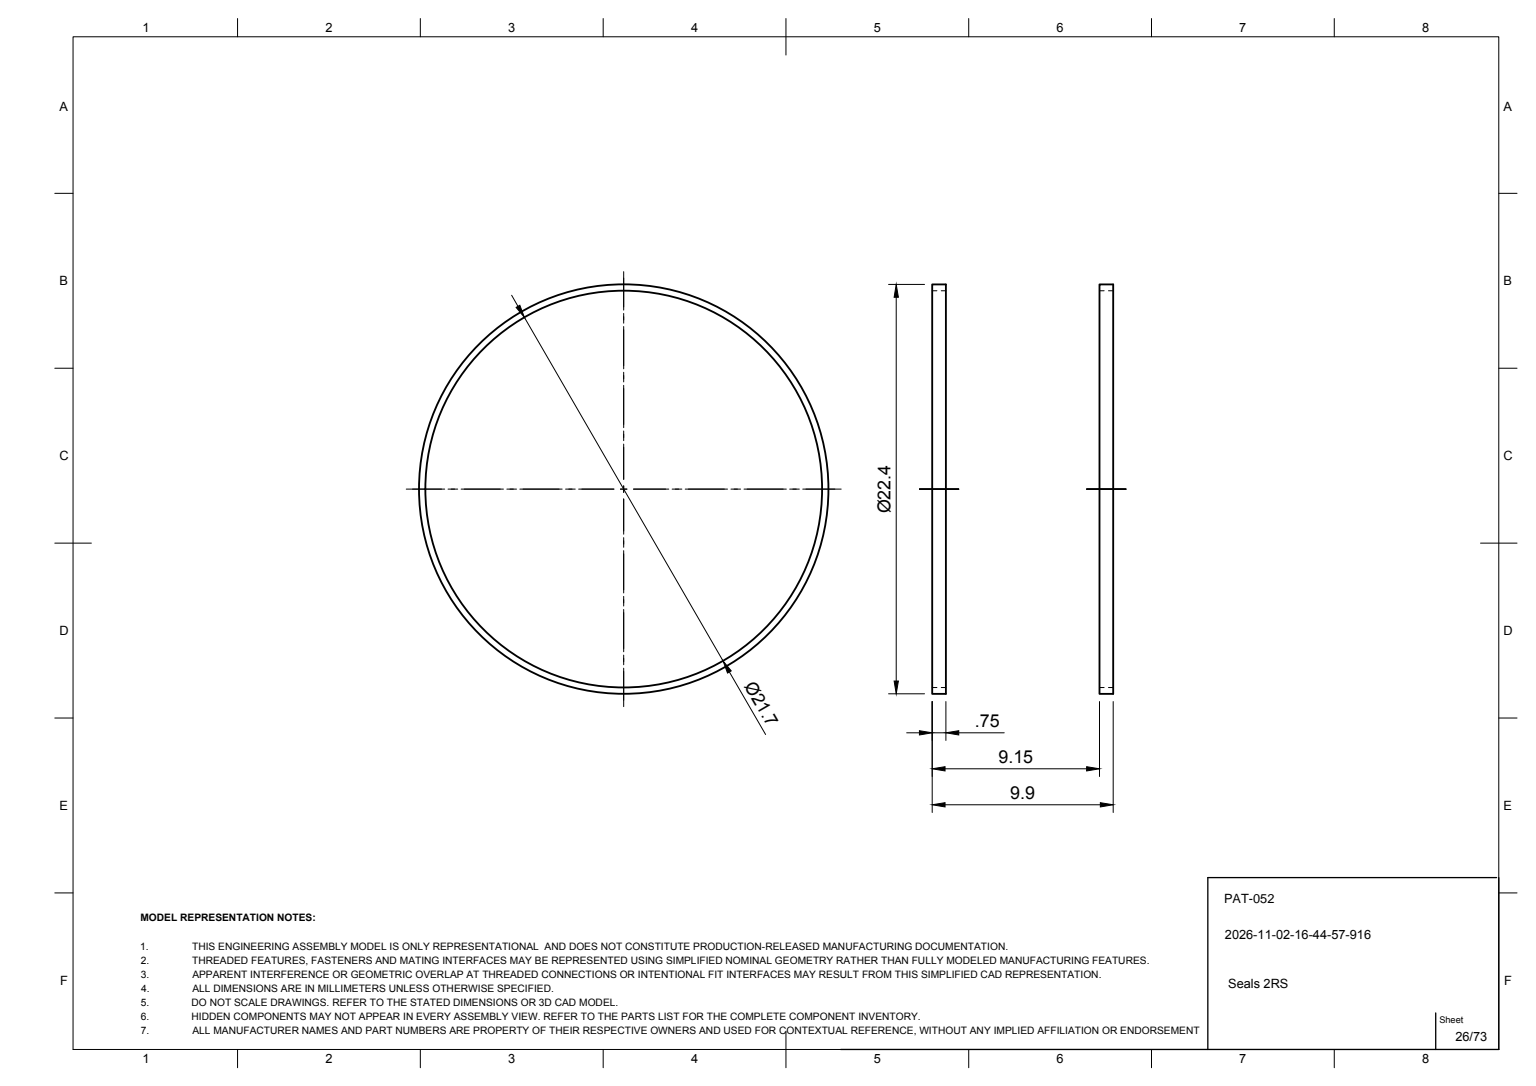
ISO-10303-21;
HEADER;
/* Generated by software containing ST-Developer
 * from STEP Tools, Inc. (www.steptools.com) 
 */

FILE_DESCRIPTION(
/* description */ ('Hand-crank gear train demonstrator'),
/* implementation_level */ '2;1');

FILE_NAME(
/* name */ 'Seals 2RS.step',
/* time_stamp */ '2026-10-28T03:22:13-07:00',
/* author */ (''),
/* organization */ (''),
/* preprocessor_version */ 'ST-DEVELOPER v20.2',
/* originating_system */ 'Autodesk Translation Framework v15.17.0.0',
/* authorisation */ '');

FILE_SCHEMA (('AUTOMOTIVE_DESIGN { 1 0 10303 214 3 1 1 }'));
ENDSEC;

DATA;
#10=MECHANICAL_DESIGN_GEOMETRIC_PRESENTATION_REPRESENTATION('',(#1210,#1211),#62758);
#1076=SHAPE_REPRESENTATION_RELATIONSHIP('SRR','None',#63049,#1140);
#1140=ADVANCED_BREP_SHAPE_REPRESENTATION('',(#1288,#1289),#62703);
#1210=STYLED_ITEM('',(#63462),#1288);
#1211=STYLED_ITEM('',(#63462),#1289);
#1288=MANIFOLD_SOLID_BREP('Body1',#16391);
#1289=MANIFOLD_SOLID_BREP('Body2',#16392);
#1492=FACE_BOUND('',#3388,.T.);
#1493=FACE_BOUND('',#3391,.T.);
#1494=FACE_BOUND('',#3394,.T.);
#1495=FACE_BOUND('',#3397,.T.);
#1694=PLANE('',#17591);
#1695=PLANE('',#17596);
#1696=PLANE('',#17599);
#1697=PLANE('',#17604);
#2301=FACE_OUTER_BOUND('',#3387,.T.);
#2302=FACE_OUTER_BOUND('',#3389,.T.);
#2303=FACE_OUTER_BOUND('',#3390,.T.);
#2304=FACE_OUTER_BOUND('',#3392,.T.);
#2305=FACE_OUTER_BOUND('',#3393,.T.);
#2306=FACE_OUTER_BOUND('',#3395,.T.);
#2307=FACE_OUTER_BOUND('',#3396,.T.);
#2308=FACE_OUTER_BOUND('',#3398,.T.);
#3387=EDGE_LOOP('',(#11633));
#3388=EDGE_LOOP('',(#11634));
#3389=EDGE_LOOP('',(#11635,#11636,#11637,#11638));
#3390=EDGE_LOOP('',(#11639));
#3391=EDGE_LOOP('',(#11640));
#3392=EDGE_LOOP('',(#11641,#11642,#11643,#11644));
#3393=EDGE_LOOP('',(#11645));
#3394=EDGE_LOOP('',(#11646));
#3395=EDGE_LOOP('',(#11647,#11648,#11649,#11650));
#3396=EDGE_LOOP('',(#11651));
#3397=EDGE_LOOP('',(#11652));
#3398=EDGE_LOOP('',(#11653,#11654,#11655,#11656));
#4435=LINE('',#24480,#5567);
#4436=LINE('',#24485,#5568);
#4437=LINE('',#24494,#5569);
#4438=LINE('',#24499,#5570);
#5567=VECTOR('',#19856,1.119765);
#5568=VECTOR('',#19863,1.085235);
#5569=VECTOR('',#19874,1.119765);
#5570=VECTOR('',#19881,1.085235);
#6786=CIRCLE('',#17592,1.119765);
#6787=CIRCLE('',#17593,1.085235);
#6788=CIRCLE('',#17595,1.119765);
#6789=CIRCLE('',#17597,1.085235);
#6790=CIRCLE('',#17600,1.119765);
#6791=CIRCLE('',#17601,1.085235);
#6792=CIRCLE('',#17603,1.119765);
#6793=CIRCLE('',#17605,1.085235);
#7485=VERTEX_POINT('',#24473);
#7486=VERTEX_POINT('',#24475);
#7487=VERTEX_POINT('',#24478);
#7488=VERTEX_POINT('',#24482);
#7489=VERTEX_POINT('',#24487);
#7490=VERTEX_POINT('',#24489);
#7491=VERTEX_POINT('',#24492);
#7492=VERTEX_POINT('',#24496);
#9068=EDGE_CURVE('',#7485,#7485,#6786,.T.);
#9069=EDGE_CURVE('',#7486,#7486,#6787,.T.);
#9070=EDGE_CURVE('',#7487,#7487,#6788,.T.);
#9071=EDGE_CURVE('',#7487,#7485,#4435,.T.);
#9072=EDGE_CURVE('',#7488,#7488,#6789,.T.);
#9073=EDGE_CURVE('',#7488,#7486,#4436,.T.);
#9074=EDGE_CURVE('',#7489,#7489,#6790,.T.);
#9075=EDGE_CURVE('',#7490,#7490,#6791,.T.);
#9076=EDGE_CURVE('',#7491,#7491,#6792,.T.);
#9077=EDGE_CURVE('',#7491,#7489,#4437,.T.);
#9078=EDGE_CURVE('',#7492,#7492,#6793,.T.);
#9079=EDGE_CURVE('',#7492,#7490,#4438,.T.);
#11633=ORIENTED_EDGE('',*,*,#9068,.F.);
#11634=ORIENTED_EDGE('',*,*,#9069,.T.);
#11635=ORIENTED_EDGE('',*,*,#9070,.F.);
#11636=ORIENTED_EDGE('',*,*,#9071,.T.);
#11637=ORIENTED_EDGE('',*,*,#9068,.T.);
#11638=ORIENTED_EDGE('',*,*,#9071,.F.);
#11639=ORIENTED_EDGE('',*,*,#9070,.T.);
#11640=ORIENTED_EDGE('',*,*,#9072,.F.);
#11641=ORIENTED_EDGE('',*,*,#9072,.T.);
#11642=ORIENTED_EDGE('',*,*,#9073,.T.);
#11643=ORIENTED_EDGE('',*,*,#9069,.F.);
#11644=ORIENTED_EDGE('',*,*,#9073,.F.);
#11645=ORIENTED_EDGE('',*,*,#9074,.F.);
#11646=ORIENTED_EDGE('',*,*,#9075,.T.);
#11647=ORIENTED_EDGE('',*,*,#9076,.F.);
#11648=ORIENTED_EDGE('',*,*,#9077,.T.);
#11649=ORIENTED_EDGE('',*,*,#9074,.T.);
#11650=ORIENTED_EDGE('',*,*,#9077,.F.);
#11651=ORIENTED_EDGE('',*,*,#9076,.T.);
#11652=ORIENTED_EDGE('',*,*,#9078,.F.);
#11653=ORIENTED_EDGE('',*,*,#9078,.T.);
#11654=ORIENTED_EDGE('',*,*,#9079,.T.);
#11655=ORIENTED_EDGE('',*,*,#9075,.F.);
#11656=ORIENTED_EDGE('',*,*,#9079,.F.);
#15261=CYLINDRICAL_SURFACE('',#17594,1.119765);
#15262=CYLINDRICAL_SURFACE('',#17598,1.085235);
#15263=CYLINDRICAL_SURFACE('',#17602,1.119765);
#15264=CYLINDRICAL_SURFACE('',#17606,1.085235);
#15611=ADVANCED_FACE('',(#2301,#1492),#1694,.T.);
#15612=ADVANCED_FACE('',(#2302),#15261,.T.);
#15613=ADVANCED_FACE('',(#2303,#1493),#1695,.T.);
#15614=ADVANCED_FACE('',(#2304),#15262,.F.);
#15615=ADVANCED_FACE('',(#2305,#1494),#1696,.T.);
#15616=ADVANCED_FACE('',(#2306),#15263,.T.);
#15617=ADVANCED_FACE('',(#2307,#1495),#1697,.T.);
#15618=ADVANCED_FACE('',(#2308),#15264,.F.);
#16391=CLOSED_SHELL('',(#15611,#15612,#15613,#15614));
#16392=CLOSED_SHELL('',(#15615,#15616,#15617,#15618));
#17590=AXIS2_PLACEMENT_3D('',#24471,#19844,#19845);
#17591=AXIS2_PLACEMENT_3D('',#24472,#19846,#19847);
#17592=AXIS2_PLACEMENT_3D('',#24474,#19848,#19849);
#17593=AXIS2_PLACEMENT_3D('',#24476,#19850,#19851);
#17594=AXIS2_PLACEMENT_3D('',#24477,#19852,#19853);
#17595=AXIS2_PLACEMENT_3D('',#24479,#19854,#19855);
#17596=AXIS2_PLACEMENT_3D('',#24481,#19857,#19858);
#17597=AXIS2_PLACEMENT_3D('',#24483,#19859,#19860);
#17598=AXIS2_PLACEMENT_3D('',#24484,#19861,#19862);
#17599=AXIS2_PLACEMENT_3D('',#24486,#19864,#19865);
#17600=AXIS2_PLACEMENT_3D('',#24488,#19866,#19867);
#17601=AXIS2_PLACEMENT_3D('',#24490,#19868,#19869);
#17602=AXIS2_PLACEMENT_3D('',#24491,#19870,#19871);
#17603=AXIS2_PLACEMENT_3D('',#24493,#19872,#19873);
#17604=AXIS2_PLACEMENT_3D('',#24495,#19875,#19876);
#17605=AXIS2_PLACEMENT_3D('',#24497,#19877,#19878);
#17606=AXIS2_PLACEMENT_3D('',#24498,#19879,#19880);
#19844=DIRECTION('axis',(0.,0.,1.));
#19845=DIRECTION('refdir',(1.,0.,0.));
#19846=DIRECTION('center_axis',(0.,1.,0.));
#19847=DIRECTION('ref_axis',(0.,0.,1.));
#19848=DIRECTION('center_axis',(0.,-1.,0.));
#19849=DIRECTION('ref_axis',(1.,0.,0.));
#19850=DIRECTION('center_axis',(0.,-1.,0.));
#19851=DIRECTION('ref_axis',(1.,0.,0.));
#19852=DIRECTION('center_axis',(0.,-1.,0.));
#19853=DIRECTION('ref_axis',(1.,0.,0.));
#19854=DIRECTION('center_axis',(0.,-1.,0.));
#19855=DIRECTION('ref_axis',(1.,0.,0.));
#19856=DIRECTION('',(0.,1.,0.));
#19857=DIRECTION('center_axis',(0.,-1.,0.));
#19858=DIRECTION('ref_axis',(0.,0.,-1.));
#19859=DIRECTION('center_axis',(0.,-1.,0.));
#19860=DIRECTION('ref_axis',(1.,0.,0.));
#19861=DIRECTION('center_axis',(0.,-1.,0.));
#19862=DIRECTION('ref_axis',(1.,0.,0.));
#19863=DIRECTION('',(0.,1.,0.));
#19864=DIRECTION('center_axis',(0.,1.,0.));
#19865=DIRECTION('ref_axis',(0.,0.,1.));
#19866=DIRECTION('center_axis',(0.,-1.,0.));
#19867=DIRECTION('ref_axis',(1.,0.,0.));
#19868=DIRECTION('center_axis',(0.,-1.,0.));
#19869=DIRECTION('ref_axis',(1.,0.,0.));
#19870=DIRECTION('center_axis',(0.,-1.,0.));
#19871=DIRECTION('ref_axis',(1.,0.,0.));
#19872=DIRECTION('center_axis',(0.,-1.,0.));
#19873=DIRECTION('ref_axis',(1.,0.,0.));
#19874=DIRECTION('',(0.,1.,0.));
#19875=DIRECTION('center_axis',(0.,-1.,0.));
#19876=DIRECTION('ref_axis',(0.,0.,-1.));
#19877=DIRECTION('center_axis',(0.,-1.,0.));
#19878=DIRECTION('ref_axis',(1.,0.,0.));
#19879=DIRECTION('center_axis',(0.,-1.,0.));
#19880=DIRECTION('ref_axis',(1.,0.,0.));
#19881=DIRECTION('',(0.,1.,0.));
#24471=CARTESIAN_POINT('',(0.,0.,0.));
#24472=CARTESIAN_POINT('Origin',(1.119765,0.495,0.));
#24473=CARTESIAN_POINT('',(-1.119765,0.495,-1.37131662304724E-16));
#24474=CARTESIAN_POINT('Origin',(0.,0.495,0.));
#24475=CARTESIAN_POINT('',(-1.085235,0.495,-1.32902956907268E-16));
#24476=CARTESIAN_POINT('Origin',(0.,0.495,0.));
#24477=CARTESIAN_POINT('Origin',(0.,0.4575,0.));
#24478=CARTESIAN_POINT('',(-1.119765,0.42,-1.37131662304724E-16));
#24479=CARTESIAN_POINT('Origin',(0.,0.42,0.));
#24480=CARTESIAN_POINT('',(-1.119765,0.4575,-1.37131662304724E-16));
#24481=CARTESIAN_POINT('Origin',(1.085235,0.42,0.));
#24482=CARTESIAN_POINT('',(-1.085235,0.42,-1.32902956907268E-16));
#24483=CARTESIAN_POINT('Origin',(0.,0.42,0.));
#24484=CARTESIAN_POINT('Origin',(0.,0.4575,0.));
#24485=CARTESIAN_POINT('',(-1.085235,0.4575,-1.32902956907268E-16));
#24486=CARTESIAN_POINT('Origin',(1.119765,-0.42,0.));
#24487=CARTESIAN_POINT('',(-1.119765,-0.42,-1.37131662304724E-16));
#24488=CARTESIAN_POINT('Origin',(0.,-0.42,0.));
#24489=CARTESIAN_POINT('',(-1.085235,-0.42,-1.32902956907268E-16));
#24490=CARTESIAN_POINT('Origin',(0.,-0.42,0.));
#24491=CARTESIAN_POINT('Origin',(0.,-0.4575,0.));
#24492=CARTESIAN_POINT('',(-1.119765,-0.495,-1.37131662304724E-16));
#24493=CARTESIAN_POINT('Origin',(0.,-0.495,0.));
#24494=CARTESIAN_POINT('',(-1.119765,-0.4575,-1.37131662304724E-16));
#24495=CARTESIAN_POINT('Origin',(1.085235,-0.495,0.));
#24496=CARTESIAN_POINT('',(-1.085235,-0.495,-1.32902956907268E-16));
#24497=CARTESIAN_POINT('Origin',(0.,-0.495,0.));
#24498=CARTESIAN_POINT('Origin',(0.,-0.4575,0.));
#24499=CARTESIAN_POINT('',(-1.085235,-0.4575,-1.32902956907268E-16));
#62629=UNCERTAINTY_MEASURE_WITH_UNIT(LENGTH_MEASURE(0.001),#62759,
'DISTANCE_ACCURACY_VALUE',
'Maximum model space distance between geometric entities at asserted c
onnectivities');
#62684=UNCERTAINTY_MEASURE_WITH_UNIT(LENGTH_MEASURE(0.001),#62759,
'DISTANCE_ACCURACY_VALUE',
'Maximum model space distance between geometric entities at asserted c
onnectivities');
#62703=(
GEOMETRIC_REPRESENTATION_CONTEXT(3)
GLOBAL_UNCERTAINTY_ASSIGNED_CONTEXT((#62629))
GLOBAL_UNIT_ASSIGNED_CONTEXT((#62759,#62761,#62762))
REPRESENTATION_CONTEXT('','3D')
);
#62758=(
GEOMETRIC_REPRESENTATION_CONTEXT(3)
GLOBAL_UNCERTAINTY_ASSIGNED_CONTEXT((#62684))
GLOBAL_UNIT_ASSIGNED_CONTEXT((#62759,#62761,#62762))
REPRESENTATION_CONTEXT('','3D')
);
#62759=(
LENGTH_UNIT()
NAMED_UNIT(*)
SI_UNIT(.CENTI.,.METRE.)
);
#62761=(
NAMED_UNIT(*)
PLANE_ANGLE_UNIT()
SI_UNIT($,.RADIAN.)
);
#62762=(
NAMED_UNIT(*)
SI_UNIT($,.STERADIAN.)
SOLID_ANGLE_UNIT()
);
#62781=SHAPE_DEFINITION_REPRESENTATION(#62854,#63049);
#62854=PRODUCT_DEFINITION_SHAPE('',$,#63123);
#63049=SHAPE_REPRESENTATION('',(#17590),#62703);
#63104=PRODUCT_DEFINITION_CONTEXT('part definition',#63325,'design');
#63123=PRODUCT_DEFINITION('Seals 2RS','Seals 2RS',#63196,#63104);
#63196=PRODUCT_DEFINITION_FORMATION('',$,#63345);
#63325=APPLICATION_CONTEXT(
'Core Data for Automotive Mechanical Design Process');
#63326=PRODUCT_CONTEXT('part definition',#63325,'mechanical');
#63345=PRODUCT('Seals 2RS','Seals 2RS','Seals 2RS',(#63326));
#63456=COLOUR_RGB('Grey',0.48,0.52,0.57);
#63457=FILL_AREA_STYLE_COLOUR('',#63456);
#63458=FILL_AREA_STYLE('',(#63457));
#63459=SURFACE_STYLE_FILL_AREA(#63458);
#63460=SURFACE_SIDE_STYLE('',(#63459));
#63461=SURFACE_STYLE_USAGE(.BOTH.,#63460);
#63462=PRESENTATION_STYLE_ASSIGNMENT((#63461));
ENDSEC;
END-ISO-10303-21;
